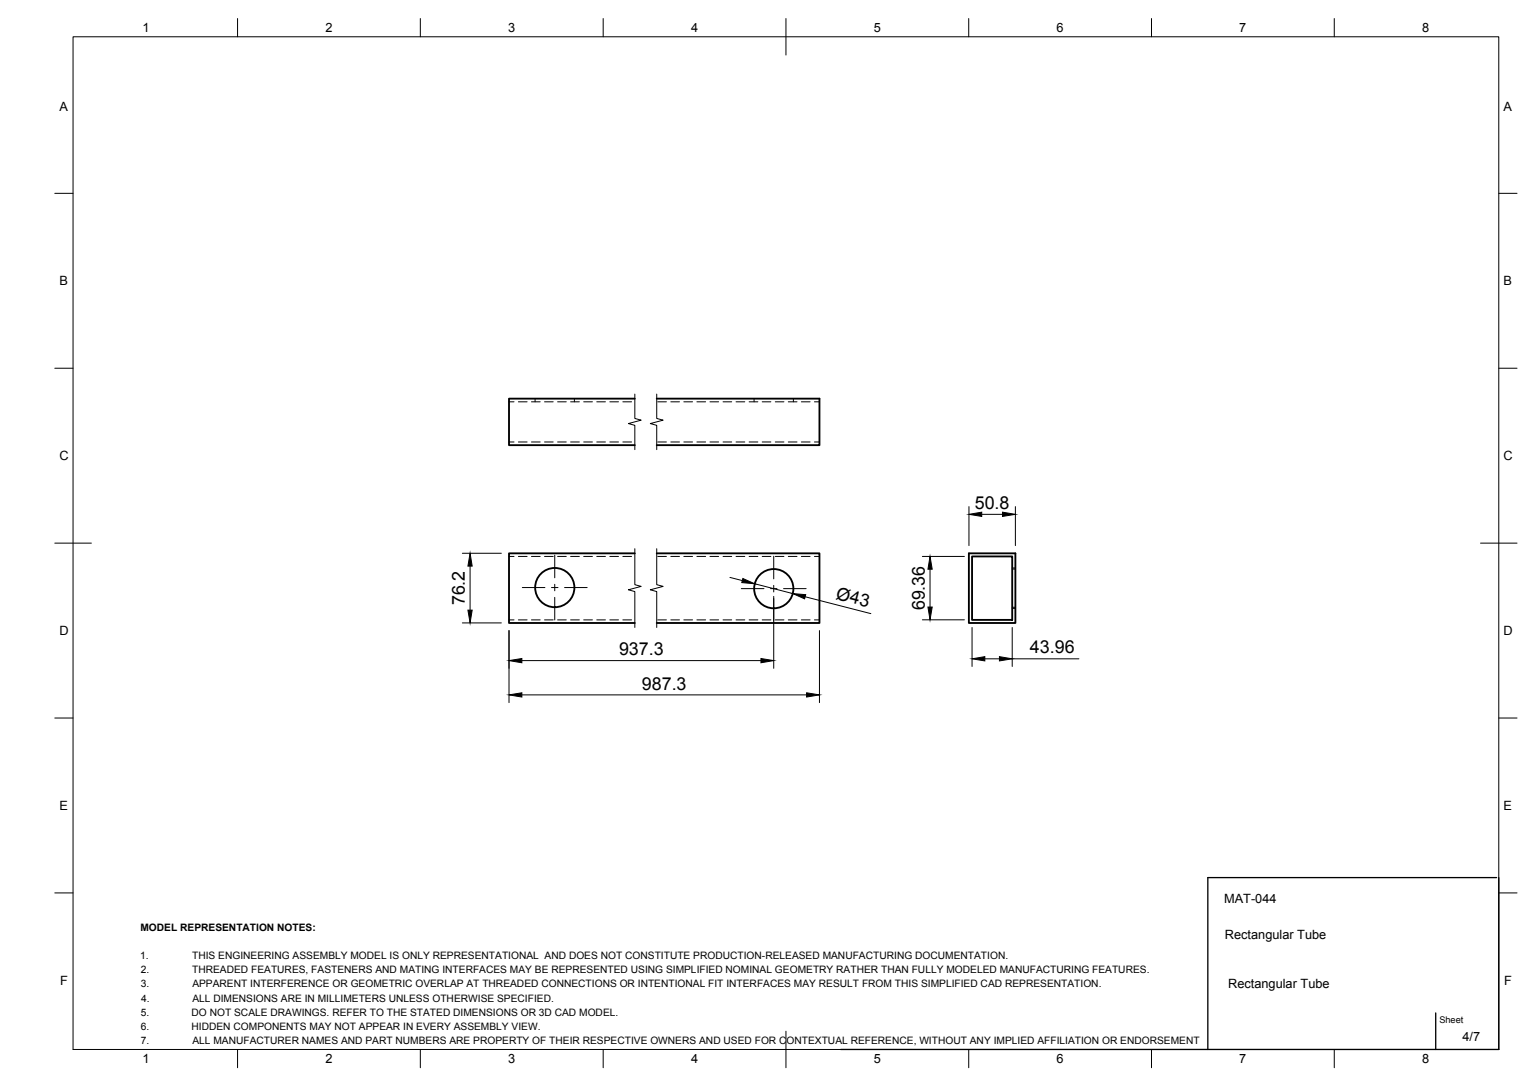
ISO-10303-21;
HEADER;
/* Generated by software containing ST-Developer
 * from STEP Tools, Inc. (www.steptools.com) 
 */

FILE_DESCRIPTION(
/* description */ ('STEP AP214'),
/* implementation_level */ '2;1');

FILE_NAME(
/* name */ 'Rectangular Tube.step',
/* time_stamp */ '2026-11-14T22:20:24-08:00',
/* author */ (''),
/* organization */ (''),
/* preprocessor_version */ 'ST-DEVELOPER v20.2',
/* originating_system */ 'Autodesk Translation Framework v15.17.0.0',
/* authorisation */ '');

FILE_SCHEMA (('AUTOMOTIVE_DESIGN { 1 0 10303 214 3 1 1 }'));
ENDSEC;

DATA;
#10=MECHANICAL_DESIGN_GEOMETRIC_PRESENTATION_REPRESENTATION('',(#83),#2794);
#73=SHAPE_REPRESENTATION_RELATIONSHIP('SRR','None',#2828,#78);
#78=ADVANCED_BREP_SHAPE_REPRESENTATION('',(#88),#2790);
#83=STYLED_ITEM('',(#2862),#88);
#88=MANIFOLD_SOLID_BREP('Body1',#1642);
#108=FACE_BOUND('',#354,.T.);
#109=FACE_BOUND('',#355,.T.);
#110=FACE_BOUND('',#362,.T.);
#111=FACE_BOUND('',#363,.T.);
#112=FACE_BOUND('',#366,.T.);
#113=FACE_BOUND('',#368,.T.);
#158=PLANE('',#1801);
#159=PLANE('',#1802);
#160=PLANE('',#1803);
#161=PLANE('',#1804);
#162=PLANE('',#1805);
#163=PLANE('',#1806);
#164=PLANE('',#1807);
#165=PLANE('',#1808);
#166=PLANE('',#1809);
#167=PLANE('',#1810);
#244=FACE_OUTER_BOUND('',#351,.T.);
#245=FACE_OUTER_BOUND('',#352,.T.);
#246=FACE_OUTER_BOUND('',#353,.T.);
#247=FACE_OUTER_BOUND('',#356,.T.);
#248=FACE_OUTER_BOUND('',#357,.T.);
#249=FACE_OUTER_BOUND('',#358,.T.);
#250=FACE_OUTER_BOUND('',#359,.T.);
#251=FACE_OUTER_BOUND('',#360,.T.);
#252=FACE_OUTER_BOUND('',#361,.T.);
#253=FACE_OUTER_BOUND('',#364,.T.);
#254=FACE_OUTER_BOUND('',#365,.T.);
#255=FACE_OUTER_BOUND('',#367,.T.);
#351=EDGE_LOOP('',(#1382,#1383,#1384,#1385));
#352=EDGE_LOOP('',(#1386,#1387,#1388,#1389));
#353=EDGE_LOOP('',(#1390,#1391,#1392,#1393));
#354=EDGE_LOOP('',(#1394));
#355=EDGE_LOOP('',(#1395));
#356=EDGE_LOOP('',(#1396,#1397,#1398,#1399));
#357=EDGE_LOOP('',(#1400,#1401,#1402,#1403));
#358=EDGE_LOOP('',(#1404,#1405,#1406,#1407));
#359=EDGE_LOOP('',(#1408,#1409,#1410,#1411));
#360=EDGE_LOOP('',(#1412,#1413,#1414,#1415));
#361=EDGE_LOOP('',(#1416,#1417,#1418,#1419));
#362=EDGE_LOOP('',(#1420));
#363=EDGE_LOOP('',(#1421));
#364=EDGE_LOOP('',(#1422,#1423,#1424,#1425));
#365=EDGE_LOOP('',(#1426,#1427,#1428,#1429));
#366=EDGE_LOOP('',(#1430,#1431,#1432,#1433));
#367=EDGE_LOOP('',(#1434,#1435,#1436,#1437));
#368=EDGE_LOOP('',(#1438,#1439,#1440,#1441));
#496=LINE('',#2611,#665);
#497=LINE('',#2617,#666);
#498=LINE('',#2622,#667);
#499=LINE('',#2624,#668);
#500=LINE('',#2626,#669);
#501=LINE('',#2627,#670);
#502=LINE('',#2630,#671);
#503=LINE('',#2632,#672);
#504=LINE('',#2633,#673);
#505=LINE('',#2636,#674);
#506=LINE('',#2638,#675);
#507=LINE('',#2639,#676);
#508=LINE('',#2643,#677);
#509=LINE('',#2645,#678);
#510=LINE('',#2647,#679);
#511=LINE('',#2648,#680);
#512=LINE('',#2651,#681);
#513=LINE('',#2653,#682);
#514=LINE('',#2654,#683);
#515=LINE('',#2657,#684);
#516=LINE('',#2659,#685);
#517=LINE('',#2660,#686);
#518=LINE('',#2662,#687);
#519=LINE('',#2663,#688);
#520=LINE('',#2665,#689);
#521=LINE('',#2666,#690);
#665=VECTOR('',#2149,21.5000000000002);
#666=VECTOR('',#2156,21.5000000000002);
#667=VECTOR('',#2161,1000.);
#668=VECTOR('',#2162,1000.);
#669=VECTOR('',#2163,1000.);
#670=VECTOR('',#2164,1000.);
#671=VECTOR('',#2167,1000.);
#672=VECTOR('',#2168,1000.);
#673=VECTOR('',#2169,1000.);
#674=VECTOR('',#2172,1000.);
#675=VECTOR('',#2173,1000.);
#676=VECTOR('',#2174,1000.);
#677=VECTOR('',#2177,1000.);
#678=VECTOR('',#2178,1000.);
#679=VECTOR('',#2179,1000.);
#680=VECTOR('',#2180,1000.);
#681=VECTOR('',#2183,1000.);
#682=VECTOR('',#2184,1000.);
#683=VECTOR('',#2185,1000.);
#684=VECTOR('',#2188,1000.);
#685=VECTOR('',#2189,1000.);
#686=VECTOR('',#2190,1000.);
#687=VECTOR('',#2193,1000.);
#688=VECTOR('',#2194,1000.);
#689=VECTOR('',#2197,1000.);
#690=VECTOR('',#2198,1000.);
#762=CIRCLE('',#1796,21.5000000000002);
#763=CIRCLE('',#1797,21.5000000000002);
#764=CIRCLE('',#1799,21.5000000000002);
#765=CIRCLE('',#1800,21.5000000000002);
#851=VERTEX_POINT('',#2608);
#852=VERTEX_POINT('',#2610);
#853=VERTEX_POINT('',#2614);
#854=VERTEX_POINT('',#2616);
#855=VERTEX_POINT('',#2620);
#856=VERTEX_POINT('',#2621);
#857=VERTEX_POINT('',#2623);
#858=VERTEX_POINT('',#2625);
#859=VERTEX_POINT('',#2629);
#860=VERTEX_POINT('',#2631);
#861=VERTEX_POINT('',#2635);
#862=VERTEX_POINT('',#2637);
#863=VERTEX_POINT('',#2641);
#864=VERTEX_POINT('',#2642);
#865=VERTEX_POINT('',#2644);
#866=VERTEX_POINT('',#2646);
#867=VERTEX_POINT('',#2650);
#868=VERTEX_POINT('',#2652);
#869=VERTEX_POINT('',#2656);
#870=VERTEX_POINT('',#2658);
#1036=EDGE_CURVE('',#851,#851,#762,.T.);
#1037=EDGE_CURVE('',#851,#852,#496,.T.);
#1038=EDGE_CURVE('',#852,#852,#763,.T.);
#1039=EDGE_CURVE('',#853,#853,#764,.T.);
#1040=EDGE_CURVE('',#853,#854,#497,.T.);
#1041=EDGE_CURVE('',#854,#854,#765,.T.);
#1042=EDGE_CURVE('',#855,#856,#498,.T.);
#1043=EDGE_CURVE('',#857,#856,#499,.T.);
#1044=EDGE_CURVE('',#858,#857,#500,.T.);
#1045=EDGE_CURVE('',#858,#855,#501,.T.);
#1046=EDGE_CURVE('',#856,#859,#502,.T.);
#1047=EDGE_CURVE('',#860,#859,#503,.T.);
#1048=EDGE_CURVE('',#857,#860,#504,.T.);
#1049=EDGE_CURVE('',#859,#861,#505,.T.);
#1050=EDGE_CURVE('',#862,#861,#506,.T.);
#1051=EDGE_CURVE('',#860,#862,#507,.T.);
#1052=EDGE_CURVE('',#863,#864,#508,.T.);
#1053=EDGE_CURVE('',#865,#863,#509,.T.);
#1054=EDGE_CURVE('',#865,#866,#510,.T.);
#1055=EDGE_CURVE('',#866,#864,#511,.T.);
#1056=EDGE_CURVE('',#867,#863,#512,.T.);
#1057=EDGE_CURVE('',#868,#867,#513,.T.);
#1058=EDGE_CURVE('',#868,#865,#514,.T.);
#1059=EDGE_CURVE('',#869,#867,#515,.T.);
#1060=EDGE_CURVE('',#870,#869,#516,.T.);
#1061=EDGE_CURVE('',#870,#868,#517,.T.);
#1062=EDGE_CURVE('',#864,#869,#518,.T.);
#1063=EDGE_CURVE('',#866,#870,#519,.T.);
#1064=EDGE_CURVE('',#861,#855,#520,.T.);
#1065=EDGE_CURVE('',#862,#858,#521,.T.);
#1382=ORIENTED_EDGE('',*,*,#1036,.T.);
#1383=ORIENTED_EDGE('',*,*,#1037,.T.);
#1384=ORIENTED_EDGE('',*,*,#1038,.T.);
#1385=ORIENTED_EDGE('',*,*,#1037,.F.);
#1386=ORIENTED_EDGE('',*,*,#1039,.T.);
#1387=ORIENTED_EDGE('',*,*,#1040,.T.);
#1388=ORIENTED_EDGE('',*,*,#1041,.T.);
#1389=ORIENTED_EDGE('',*,*,#1040,.F.);
#1390=ORIENTED_EDGE('',*,*,#1042,.T.);
#1391=ORIENTED_EDGE('',*,*,#1043,.F.);
#1392=ORIENTED_EDGE('',*,*,#1044,.F.);
#1393=ORIENTED_EDGE('',*,*,#1045,.T.);
#1394=ORIENTED_EDGE('',*,*,#1038,.F.);
#1395=ORIENTED_EDGE('',*,*,#1041,.F.);
#1396=ORIENTED_EDGE('',*,*,#1046,.T.);
#1397=ORIENTED_EDGE('',*,*,#1047,.F.);
#1398=ORIENTED_EDGE('',*,*,#1048,.F.);
#1399=ORIENTED_EDGE('',*,*,#1043,.T.);
#1400=ORIENTED_EDGE('',*,*,#1049,.T.);
#1401=ORIENTED_EDGE('',*,*,#1050,.F.);
#1402=ORIENTED_EDGE('',*,*,#1051,.F.);
#1403=ORIENTED_EDGE('',*,*,#1047,.T.);
#1404=ORIENTED_EDGE('',*,*,#1052,.F.);
#1405=ORIENTED_EDGE('',*,*,#1053,.F.);
#1406=ORIENTED_EDGE('',*,*,#1054,.T.);
#1407=ORIENTED_EDGE('',*,*,#1055,.T.);
#1408=ORIENTED_EDGE('',*,*,#1056,.F.);
#1409=ORIENTED_EDGE('',*,*,#1057,.F.);
#1410=ORIENTED_EDGE('',*,*,#1058,.T.);
#1411=ORIENTED_EDGE('',*,*,#1053,.T.);
#1412=ORIENTED_EDGE('',*,*,#1059,.F.);
#1413=ORIENTED_EDGE('',*,*,#1060,.F.);
#1414=ORIENTED_EDGE('',*,*,#1061,.T.);
#1415=ORIENTED_EDGE('',*,*,#1057,.T.);
#1416=ORIENTED_EDGE('',*,*,#1062,.F.);
#1417=ORIENTED_EDGE('',*,*,#1055,.F.);
#1418=ORIENTED_EDGE('',*,*,#1063,.T.);
#1419=ORIENTED_EDGE('',*,*,#1060,.T.);
#1420=ORIENTED_EDGE('',*,*,#1036,.F.);
#1421=ORIENTED_EDGE('',*,*,#1039,.F.);
#1422=ORIENTED_EDGE('',*,*,#1064,.T.);
#1423=ORIENTED_EDGE('',*,*,#1045,.F.);
#1424=ORIENTED_EDGE('',*,*,#1065,.F.);
#1425=ORIENTED_EDGE('',*,*,#1050,.T.);
#1426=ORIENTED_EDGE('',*,*,#1044,.T.);
#1427=ORIENTED_EDGE('',*,*,#1048,.T.);
#1428=ORIENTED_EDGE('',*,*,#1051,.T.);
#1429=ORIENTED_EDGE('',*,*,#1065,.T.);
#1430=ORIENTED_EDGE('',*,*,#1054,.F.);
#1431=ORIENTED_EDGE('',*,*,#1058,.F.);
#1432=ORIENTED_EDGE('',*,*,#1061,.F.);
#1433=ORIENTED_EDGE('',*,*,#1063,.F.);
#1434=ORIENTED_EDGE('',*,*,#1042,.F.);
#1435=ORIENTED_EDGE('',*,*,#1064,.F.);
#1436=ORIENTED_EDGE('',*,*,#1049,.F.);
#1437=ORIENTED_EDGE('',*,*,#1046,.F.);
#1438=ORIENTED_EDGE('',*,*,#1052,.T.);
#1439=ORIENTED_EDGE('',*,*,#1062,.T.);
#1440=ORIENTED_EDGE('',*,*,#1059,.T.);
#1441=ORIENTED_EDGE('',*,*,#1056,.T.);
#1546=CYLINDRICAL_SURFACE('',#1795,21.5000000000002);
#1547=CYLINDRICAL_SURFACE('',#1798,21.5000000000002);
#1608=ADVANCED_FACE('',(#244),#1546,.F.);
#1609=ADVANCED_FACE('',(#245),#1547,.F.);
#1610=ADVANCED_FACE('',(#246,#108,#109),#158,.F.);
#1611=ADVANCED_FACE('',(#247),#159,.F.);
#1612=ADVANCED_FACE('',(#248),#160,.F.);
#1613=ADVANCED_FACE('',(#249),#161,.T.);
#1614=ADVANCED_FACE('',(#250),#162,.T.);
#1615=ADVANCED_FACE('',(#251),#163,.T.);
#1616=ADVANCED_FACE('',(#252,#110,#111),#164,.T.);
#1617=ADVANCED_FACE('',(#253),#165,.F.);
#1618=ADVANCED_FACE('',(#254,#112),#166,.T.);
#1619=ADVANCED_FACE('',(#255,#113),#167,.F.);
#1642=CLOSED_SHELL('',(#1608,#1609,#1610,#1611,#1612,#1613,#1614,#1615,
#1616,#1617,#1618,#1619));
#1794=AXIS2_PLACEMENT_3D('',#2606,#2143,#2144);
#1795=AXIS2_PLACEMENT_3D('',#2607,#2145,#2146);
#1796=AXIS2_PLACEMENT_3D('',#2609,#2147,#2148);
#1797=AXIS2_PLACEMENT_3D('',#2612,#2150,#2151);
#1798=AXIS2_PLACEMENT_3D('',#2613,#2152,#2153);
#1799=AXIS2_PLACEMENT_3D('',#2615,#2154,#2155);
#1800=AXIS2_PLACEMENT_3D('',#2618,#2157,#2158);
#1801=AXIS2_PLACEMENT_3D('',#2619,#2159,#2160);
#1802=AXIS2_PLACEMENT_3D('',#2628,#2165,#2166);
#1803=AXIS2_PLACEMENT_3D('',#2634,#2170,#2171);
#1804=AXIS2_PLACEMENT_3D('',#2640,#2175,#2176);
#1805=AXIS2_PLACEMENT_3D('',#2649,#2181,#2182);
#1806=AXIS2_PLACEMENT_3D('',#2655,#2186,#2187);
#1807=AXIS2_PLACEMENT_3D('',#2661,#2191,#2192);
#1808=AXIS2_PLACEMENT_3D('',#2664,#2195,#2196);
#1809=AXIS2_PLACEMENT_3D('',#2667,#2199,#2200);
#1810=AXIS2_PLACEMENT_3D('',#2668,#2201,#2202);
#2143=DIRECTION('axis',(0.,0.,1.));
#2144=DIRECTION('refdir',(1.,0.,0.));
#2145=DIRECTION('center_axis',(-1.,1.35175512935379E-29,1.36592399683213E-16));
#2146=DIRECTION('ref_axis',(1.36592399683213E-16,3.34927423218511E-46,1.));
#2147=DIRECTION('center_axis',(1.,-1.35175512935379E-29,-1.00041722951373E-16));
#2148=DIRECTION('ref_axis',(-1.00041722951373E-16,-8.29003070754679E-46,
-1.));
#2149=DIRECTION('',(-1.,1.35175512935379E-29,1.36592399683213E-16));
#2150=DIRECTION('center_axis',(-1.,1.35175512935379E-29,1.36592399683213E-16));
#2151=DIRECTION('ref_axis',(1.36592399683213E-16,3.34927423218511E-46,1.));
#2152=DIRECTION('center_axis',(-1.,1.35175512935379E-29,1.36592399683213E-16));
#2153=DIRECTION('ref_axis',(1.36592399683213E-16,3.34927423218511E-46,1.));
#2154=DIRECTION('center_axis',(1.,-1.35175512935379E-29,-1.00041722951373E-16));
#2155=DIRECTION('ref_axis',(-1.00041722951373E-16,-8.29003070754679E-46,
-1.));
#2156=DIRECTION('',(-1.,1.35175512935379E-29,1.36592399683213E-16));
#2157=DIRECTION('center_axis',(-1.,1.35175512935379E-29,1.36592399683213E-16));
#2158=DIRECTION('ref_axis',(1.36592399683213E-16,3.34927423218511E-46,1.));
#2159=DIRECTION('center_axis',(1.,-1.35175512935379E-29,-1.36592399683213E-16));
#2160=DIRECTION('ref_axis',(-1.36592399683213E-16,-2.26327091223021E-30,
-1.));
#2161=DIRECTION('',(1.36592399683213E-16,2.26327091223021E-30,1.));
#2162=DIRECTION('',(1.3517551293538E-29,-1.,-2.26327091223024E-30));
#2163=DIRECTION('',(1.36592399683213E-16,2.26327091223021E-30,1.));
#2164=DIRECTION('',(1.3517551293538E-29,-1.,-2.26327091223024E-30));
#2165=DIRECTION('center_axis',(-1.36592399683213E-16,-2.26327091223021E-30,
-1.));
#2166=DIRECTION('ref_axis',(-1.,1.35175512935379E-29,1.36592399683213E-16));
#2167=DIRECTION('',(1.,-1.35175512935379E-29,-1.36592399683213E-16));
#2168=DIRECTION('',(1.3517551293538E-29,-1.,-2.26327091223024E-30));
#2169=DIRECTION('',(1.,-1.35175512935379E-29,-1.36592399683213E-16));
#2170=DIRECTION('center_axis',(-1.,1.35175512935379E-29,4.55307998944045E-17));
#2171=DIRECTION('ref_axis',(4.55307998944045E-17,2.26327091223021E-30,1.));
#2172=DIRECTION('',(-4.55307998944045E-17,-2.26327091223021E-30,-1.));
#2173=DIRECTION('',(1.3517551293538E-29,-1.,-2.26327091223024E-30));
#2174=DIRECTION('',(-4.55307998944045E-17,-2.26327091223021E-30,-1.));
#2175=DIRECTION('center_axis',(1.57845630207171E-16,2.26327091223021E-30,
1.));
#2176=DIRECTION('ref_axis',(1.,-1.35175512935379E-29,-1.57845630207171E-16));
#2177=DIRECTION('',(-1.,1.35175512935379E-29,1.57845630207171E-16));
#2178=DIRECTION('',(1.3517551293538E-29,-1.,-2.26327091223024E-30));
#2179=DIRECTION('',(-1.,1.35175512935379E-29,1.57845630207171E-16));
#2180=DIRECTION('',(1.3517551293538E-29,-1.,-2.26327091223024E-30));
#2181=DIRECTION('center_axis',(-1.,1.35175512935379E-29,2.00083445902746E-16));
#2182=DIRECTION('ref_axis',(2.00083445902746E-16,2.26327091223021E-30,1.));
#2183=DIRECTION('',(-2.00083445902746E-16,-2.26327091223021E-30,-1.));
#2184=DIRECTION('',(1.3517551293538E-29,-1.,-2.26327091223024E-30));
#2185=DIRECTION('',(-2.00083445902746E-16,-2.26327091223021E-30,-1.));
#2186=DIRECTION('center_axis',(-1.57845630207171E-16,-2.26327091223021E-30,
-1.));
#2187=DIRECTION('ref_axis',(-1.,1.35175512935379E-29,1.57845630207171E-16));
#2188=DIRECTION('',(1.,-1.35175512935379E-29,-1.57845630207171E-16));
#2189=DIRECTION('',(1.3517551293538E-29,-1.,-2.26327091223024E-30));
#2190=DIRECTION('',(1.,-1.35175512935379E-29,-1.57845630207171E-16));
#2191=DIRECTION('center_axis',(1.,-1.35175512935379E-29,-1.00041722951373E-16));
#2192=DIRECTION('ref_axis',(-1.00041722951373E-16,-2.26327091223021E-30,
-1.));
#2193=DIRECTION('',(1.00041722951373E-16,2.26327091223021E-30,1.));
#2194=DIRECTION('',(1.00041722951373E-16,2.26327091223021E-30,1.));
#2195=DIRECTION('center_axis',(1.36592399683213E-16,2.26327091223021E-30,
1.));
#2196=DIRECTION('ref_axis',(1.,-1.35175512935379E-29,-1.36592399683213E-16));
#2197=DIRECTION('',(-1.,1.35175512935379E-29,1.36592399683213E-16));
#2198=DIRECTION('',(-1.,1.35175512935379E-29,1.36592399683213E-16));
#2199=DIRECTION('center_axis',(-1.3517551293538E-29,1.,-2.26327091223021E-30));
#2200=DIRECTION('ref_axis',(-1.72563323017094E-31,2.26327091223021E-30,
1.));
#2201=DIRECTION('center_axis',(-1.3517551293538E-29,1.,-2.26327091223021E-30));
#2202=DIRECTION('ref_axis',(-1.72563323017094E-31,2.26327091223021E-30,
1.));
#2606=CARTESIAN_POINT('',(0.,0.,0.));
#2607=CARTESIAN_POINT('Origin',(-15.4000000000002,937.3,0.600000000000211));
#2608=CARTESIAN_POINT('',(-21.9800000000002,937.3,-20.9));
#2609=CARTESIAN_POINT('Origin',(-21.9800000000002,937.3,0.600000000000211));
#2610=CARTESIAN_POINT('',(-25.4000000000003,937.3,-20.9));
#2611=CARTESIAN_POINT('',(-15.4000000000002,937.3,-20.9));
#2612=CARTESIAN_POINT('Origin',(-25.4000000000003,937.3,0.600000000000211));
#2613=CARTESIAN_POINT('Origin',(-15.4000000000002,50.,-0.6000000000001));
#2614=CARTESIAN_POINT('',(-21.9800000000002,50.,-22.1000000000003));
#2615=CARTESIAN_POINT('Origin',(-21.9800000000002,50.,-0.6000000000001));
#2616=CARTESIAN_POINT('',(-25.4000000000003,50.,-22.1000000000003));
#2617=CARTESIAN_POINT('',(-15.4000000000002,50.,-22.1000000000003));
#2618=CARTESIAN_POINT('Origin',(-25.4000000000003,50.,-0.6000000000001));
#2619=CARTESIAN_POINT('Origin',(-25.4000000000003,987.3,38.1000000000007));
#2620=CARTESIAN_POINT('',(-25.4000000000003,0.,-38.1000000000009));
#2621=CARTESIAN_POINT('',(-25.4000000000003,0.,38.1000000000007));
#2622=CARTESIAN_POINT('',(-25.4000000000003,0.,38.1000000000007));
#2623=CARTESIAN_POINT('',(-25.4000000000003,987.3,38.1000000000007));
#2624=CARTESIAN_POINT('',(-25.4000000000003,987.3,38.1000000000007));
#2625=CARTESIAN_POINT('',(-25.4000000000003,987.3,-38.1000000000009));
#2626=CARTESIAN_POINT('',(-25.4000000000003,987.3,38.1000000000007));
#2627=CARTESIAN_POINT('',(-25.4000000000003,987.3,-38.1000000000009));
#2628=CARTESIAN_POINT('Origin',(-25.4000000000003,987.3,38.1000000000007));
#2629=CARTESIAN_POINT('',(25.4000000000006,0.,38.1000000000014));
#2630=CARTESIAN_POINT('',(-25.4000000000003,0.,38.1000000000007));
#2631=CARTESIAN_POINT('',(25.4000000000006,987.3,38.1000000000014));
#2632=CARTESIAN_POINT('',(25.4000000000006,987.3,38.1000000000014));
#2633=CARTESIAN_POINT('',(-25.4000000000003,987.3,38.1000000000007));
#2634=CARTESIAN_POINT('Origin',(25.4000000000006,987.3,-38.1000000000007));
#2635=CARTESIAN_POINT('',(25.4000000000006,0.,-38.1000000000007));
#2636=CARTESIAN_POINT('',(25.4000000000006,0.,-38.1000000000007));
#2637=CARTESIAN_POINT('',(25.4000000000006,987.3,-38.1000000000007));
#2638=CARTESIAN_POINT('',(25.4000000000006,987.3,-38.1000000000007));
#2639=CARTESIAN_POINT('',(25.4000000000006,987.3,-38.1000000000007));
#2640=CARTESIAN_POINT('Origin',(21.9800000000002,987.3,-34.6800000000007));
#2641=CARTESIAN_POINT('',(21.9800000000002,0.,-34.6800000000007));
#2642=CARTESIAN_POINT('',(-21.9800000000002,0.,-34.6800000000009));
#2643=CARTESIAN_POINT('',(21.9800000000002,0.,-34.6800000000007));
#2644=CARTESIAN_POINT('',(21.9800000000002,987.3,-34.6800000000007));
#2645=CARTESIAN_POINT('',(21.9800000000002,987.3,-34.6800000000007));
#2646=CARTESIAN_POINT('',(-21.9800000000002,987.3,-34.6800000000009));
#2647=CARTESIAN_POINT('',(21.9800000000002,987.3,-34.6800000000007));
#2648=CARTESIAN_POINT('',(-21.9800000000002,987.3,-34.6800000000009));
#2649=CARTESIAN_POINT('Origin',(21.9800000000002,987.3,-34.6800000000007));
#2650=CARTESIAN_POINT('',(21.9800000000003,0.,34.6800000000014));
#2651=CARTESIAN_POINT('',(21.9800000000002,0.,-34.6800000000007));
#2652=CARTESIAN_POINT('',(21.9800000000003,987.3,34.6800000000014));
#2653=CARTESIAN_POINT('',(21.9800000000003,987.3,34.6800000000014));
#2654=CARTESIAN_POINT('',(21.9800000000002,987.3,-34.6800000000007));
#2655=CARTESIAN_POINT('Origin',(-21.9800000000001,987.3,34.6800000000008));
#2656=CARTESIAN_POINT('',(-21.9800000000001,0.,34.6800000000008));
#2657=CARTESIAN_POINT('',(-21.9800000000001,0.,34.6800000000008));
#2658=CARTESIAN_POINT('',(-21.9800000000001,987.3,34.6800000000008));
#2659=CARTESIAN_POINT('',(-21.9800000000001,987.3,34.6800000000008));
#2660=CARTESIAN_POINT('',(-21.9800000000001,987.3,34.6800000000008));
#2661=CARTESIAN_POINT('Origin',(-21.9800000000001,987.3,34.6800000000008));
#2662=CARTESIAN_POINT('',(-21.9800000000001,0.,34.6800000000008));
#2663=CARTESIAN_POINT('',(-21.9800000000001,987.3,34.6800000000008));
#2664=CARTESIAN_POINT('Origin',(25.4000000000006,987.3,-38.1000000000007));
#2665=CARTESIAN_POINT('',(25.4000000000006,0.,-38.1000000000007));
#2666=CARTESIAN_POINT('',(25.4000000000006,987.3,-38.1000000000007));
#2667=CARTESIAN_POINT('Origin',(0.,987.3,0.));
#2668=CARTESIAN_POINT('Origin',(0.,0.,0.));
#2783=UNCERTAINTY_MEASURE_WITH_UNIT(LENGTH_MEASURE(0.01),#2795,
'DISTANCE_ACCURACY_VALUE',
'Maximum model space distance between geometric entities at asserted c
onnectivities');
#2787=UNCERTAINTY_MEASURE_WITH_UNIT(LENGTH_MEASURE(0.01),#2795,
'DISTANCE_ACCURACY_VALUE',
'Maximum model space distance between geometric entities at asserted c
onnectivities');
#2790=(
GEOMETRIC_REPRESENTATION_CONTEXT(3)
GLOBAL_UNCERTAINTY_ASSIGNED_CONTEXT((#2783))
GLOBAL_UNIT_ASSIGNED_CONTEXT((#2795,#2797,#2798))
REPRESENTATION_CONTEXT('','3D')
);
#2794=(
GEOMETRIC_REPRESENTATION_CONTEXT(3)
GLOBAL_UNCERTAINTY_ASSIGNED_CONTEXT((#2787))
GLOBAL_UNIT_ASSIGNED_CONTEXT((#2795,#2797,#2798))
REPRESENTATION_CONTEXT('','3D')
);
#2795=(
LENGTH_UNIT()
NAMED_UNIT(*)
SI_UNIT(.MILLI.,.METRE.)
);
#2797=(
NAMED_UNIT(*)
PLANE_ANGLE_UNIT()
SI_UNIT($,.RADIAN.)
);
#2798=(
NAMED_UNIT(*)
SI_UNIT($,.STERADIAN.)
SOLID_ANGLE_UNIT()
);
#2801=SHAPE_DEFINITION_REPRESENTATION(#2807,#2828);
#2807=PRODUCT_DEFINITION_SHAPE('',$,#2835);
#2828=SHAPE_REPRESENTATION('',(#1794),#2790);
#2832=PRODUCT_DEFINITION_CONTEXT('part definition',#2852,'design');
#2835=PRODUCT_DEFINITION('Rectangular Tube','Rectangular Tube',#2841,#2832);
#2841=PRODUCT_DEFINITION_FORMATION('',$,#2856);
#2852=APPLICATION_CONTEXT(
'Core Data for Automotive Mechanical Design Process');
#2853=PRODUCT_CONTEXT('part definition',#2852,'mechanical');
#2856=PRODUCT('Rectangular Tube','Rectangular Tube',$,(#2853));
#2862=PRESENTATION_STYLE_ASSIGNMENT((#2866));
#2866=SURFACE_STYLE_USAGE(.BOTH.,#2870);
#2870=SURFACE_SIDE_STYLE('',(#2874));
#2874=SURFACE_STYLE_FILL_AREA(#2878);
#2878=FILL_AREA_STYLE('Opaque(61,176,222)',(#2882));
#2882=FILL_AREA_STYLE_COLOUR('Opaque(61,176,222)',#2886);
#2886=COLOUR_RGB('Opaque(61,176,222)',0.23921568627451,0.690196078431373,
0.870588235294118);
ENDSEC;
END-ISO-10303-21;
